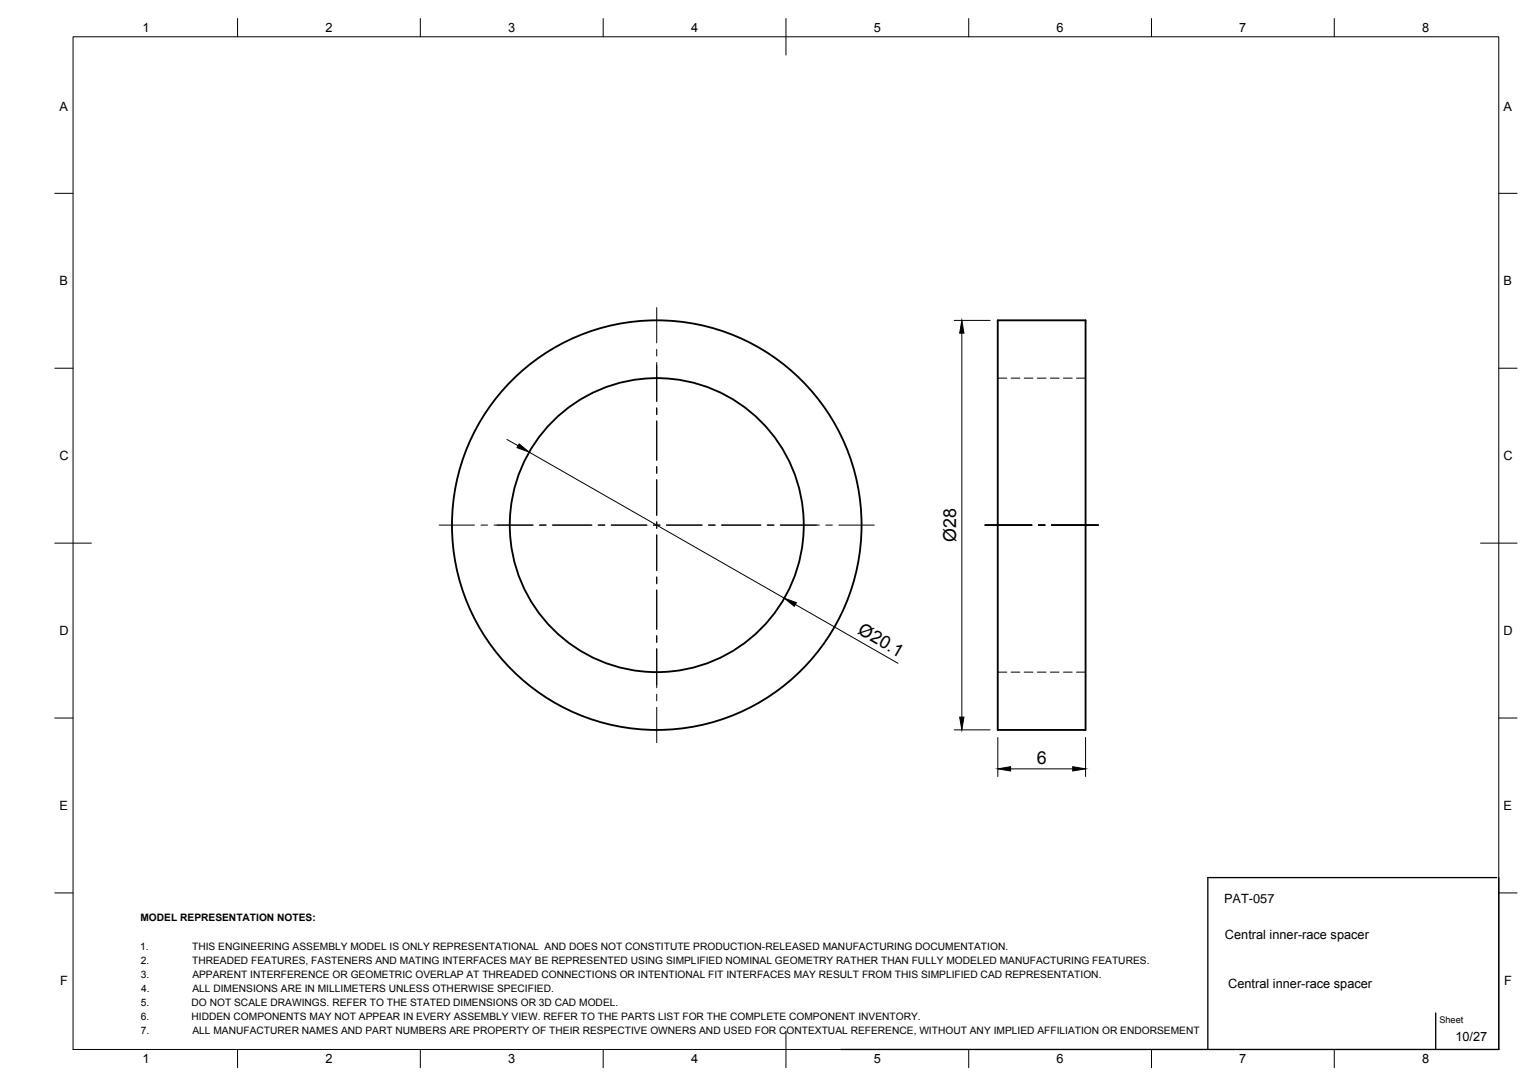
ISO-10303-21;
HEADER;
/* Generated by software containing ST-Developer
 * from STEP Tools, Inc. (www.steptools.com) 
 */

FILE_DESCRIPTION(
/* description */ ('Bearing-mounted hook block'),
/* implementation_level */ '2;1');

FILE_NAME(
/* name */ 'Central inner-race spacer.step',
/* time_stamp */ '2026-10-28T22:30:11-07:00',
/* author */ (''),
/* organization */ (''),
/* preprocessor_version */ 'ST-DEVELOPER v20.2',
/* originating_system */ 'Autodesk Translation Framework v15.17.0.0',
/* authorisation */ '');

FILE_SCHEMA (('AUTOMOTIVE_DESIGN { 1 0 10303 214 3 1 1 }'));
ENDSEC;

DATA;
#10=MECHANICAL_DESIGN_GEOMETRIC_PRESENTATION_REPRESENTATION('',(#328),#7609);
#280=SHAPE_REPRESENTATION_RELATIONSHIP('SRR','None',#7727,#304);
#304=ADVANCED_BREP_SHAPE_REPRESENTATION('',(#360),#7587);
#328=STYLED_ITEM('',(#7917),#360);
#360=MANIFOLD_SOLID_BREP('Body1',#3924);
#447=LINE('',#6319,#677);
#448=LINE('',#6325,#678);
#677=VECTOR('',#5046,1.005);
#678=VECTOR('',#5053,1.4);
#867=CYLINDRICAL_SURFACE('',#4330,1.005);
#868=CYLINDRICAL_SURFACE('',#4333,1.4);
#947=FACE_BOUND('',#1315,.T.);
#948=FACE_BOUND('',#1317,.T.);
#1050=FACE_OUTER_BOUND('',#1312,.T.);
#1051=FACE_OUTER_BOUND('',#1313,.T.);
#1052=FACE_OUTER_BOUND('',#1314,.T.);
#1053=FACE_OUTER_BOUND('',#1316,.T.);
#1312=EDGE_LOOP('',(#2824,#2825,#2826,#2827));
#1313=EDGE_LOOP('',(#2828,#2829,#2830,#2831));
#1314=EDGE_LOOP('',(#2832));
#1315=EDGE_LOOP('',(#2833));
#1316=EDGE_LOOP('',(#2834));
#1317=EDGE_LOOP('',(#2835));
#1607=CIRCLE('',#4331,1.005);
#1608=CIRCLE('',#4332,1.005);
#1609=CIRCLE('',#4334,1.4);
#1610=CIRCLE('',#4335,1.4);
#1856=VERTEX_POINT('',#6316);
#1857=VERTEX_POINT('',#6318);
#1858=VERTEX_POINT('',#6322);
#1859=VERTEX_POINT('',#6324);
#2222=EDGE_CURVE('',#1856,#1856,#1607,.T.);
#2223=EDGE_CURVE('',#1856,#1857,#447,.T.);
#2224=EDGE_CURVE('',#1857,#1857,#1608,.T.);
#2225=EDGE_CURVE('',#1858,#1858,#1609,.T.);
#2226=EDGE_CURVE('',#1858,#1859,#448,.T.);
#2227=EDGE_CURVE('',#1859,#1859,#1610,.T.);
#2824=ORIENTED_EDGE('',*,*,#2222,.F.);
#2825=ORIENTED_EDGE('',*,*,#2223,.T.);
#2826=ORIENTED_EDGE('',*,*,#2224,.T.);
#2827=ORIENTED_EDGE('',*,*,#2223,.F.);
#2828=ORIENTED_EDGE('',*,*,#2225,.F.);
#2829=ORIENTED_EDGE('',*,*,#2226,.T.);
#2830=ORIENTED_EDGE('',*,*,#2227,.T.);
#2831=ORIENTED_EDGE('',*,*,#2226,.F.);
#2832=ORIENTED_EDGE('',*,*,#2225,.T.);
#2833=ORIENTED_EDGE('',*,*,#2222,.T.);
#2834=ORIENTED_EDGE('',*,*,#2227,.F.);
#2835=ORIENTED_EDGE('',*,*,#2224,.F.);
#3586=PLANE('',#4336);
#3587=PLANE('',#4337);
#3732=ADVANCED_FACE('',(#1050),#867,.F.);
#3733=ADVANCED_FACE('',(#1051),#868,.T.);
#3734=ADVANCED_FACE('',(#1052,#947),#3586,.T.);
#3735=ADVANCED_FACE('',(#1053,#948),#3587,.F.);
#3924=CLOSED_SHELL('',(#3732,#3733,#3734,#3735));
#4329=AXIS2_PLACEMENT_3D('',#6314,#5040,#5041);
#4330=AXIS2_PLACEMENT_3D('',#6315,#5042,#5043);
#4331=AXIS2_PLACEMENT_3D('',#6317,#5044,#5045);
#4332=AXIS2_PLACEMENT_3D('',#6320,#5047,#5048);
#4333=AXIS2_PLACEMENT_3D('',#6321,#5049,#5050);
#4334=AXIS2_PLACEMENT_3D('',#6323,#5051,#5052);
#4335=AXIS2_PLACEMENT_3D('',#6326,#5054,#5055);
#4336=AXIS2_PLACEMENT_3D('',#6327,#5056,#5057);
#4337=AXIS2_PLACEMENT_3D('',#6328,#5058,#5059);
#5040=DIRECTION('axis',(0.,0.,1.));
#5041=DIRECTION('refdir',(1.,0.,0.));
#5042=DIRECTION('center_axis',(0.,1.,0.));
#5043=DIRECTION('ref_axis',(1.,0.,0.));
#5044=DIRECTION('center_axis',(0.,-1.,0.));
#5045=DIRECTION('ref_axis',(1.,0.,0.));
#5046=DIRECTION('',(0.,-1.,0.));
#5047=DIRECTION('center_axis',(0.,-1.,0.));
#5048=DIRECTION('ref_axis',(1.,0.,0.));
#5049=DIRECTION('center_axis',(0.,1.,0.));
#5050=DIRECTION('ref_axis',(1.,0.,0.));
#5051=DIRECTION('center_axis',(0.,1.,0.));
#5052=DIRECTION('ref_axis',(1.,0.,0.));
#5053=DIRECTION('',(0.,-1.,0.));
#5054=DIRECTION('center_axis',(0.,1.,0.));
#5055=DIRECTION('ref_axis',(1.,0.,0.));
#5056=DIRECTION('center_axis',(0.,1.,0.));
#5057=DIRECTION('ref_axis',(1.,0.,0.));
#5058=DIRECTION('center_axis',(0.,1.,0.));
#5059=DIRECTION('ref_axis',(1.,0.,0.));
#6314=CARTESIAN_POINT('',(0.,0.,0.));
#6315=CARTESIAN_POINT('Origin',(0.,-0.3,12.));
#6316=CARTESIAN_POINT('',(-1.005,0.3,12.));
#6317=CARTESIAN_POINT('Origin',(0.,0.3,12.));
#6318=CARTESIAN_POINT('',(-1.005,-0.3,12.));
#6319=CARTESIAN_POINT('',(-1.005,-0.3,12.));
#6320=CARTESIAN_POINT('Origin',(0.,-0.3,12.));
#6321=CARTESIAN_POINT('Origin',(0.,-0.3,12.));
#6322=CARTESIAN_POINT('',(-1.4,0.3,12.));
#6323=CARTESIAN_POINT('Origin',(0.,0.3,12.));
#6324=CARTESIAN_POINT('',(-1.4,-0.3,12.));
#6325=CARTESIAN_POINT('',(-1.4,-0.3,12.));
#6326=CARTESIAN_POINT('Origin',(0.,-0.3,12.));
#6327=CARTESIAN_POINT('Origin',(0.,0.3,12.));
#6328=CARTESIAN_POINT('Origin',(0.,-0.3,12.));
#7557=UNCERTAINTY_MEASURE_WITH_UNIT(LENGTH_MEASURE(0.001),#7610,
'DISTANCE_ACCURACY_VALUE',
'Maximum model space distance between geometric entities at asserted c
onnectivities');
#7579=UNCERTAINTY_MEASURE_WITH_UNIT(LENGTH_MEASURE(0.001),#7610,
'DISTANCE_ACCURACY_VALUE',
'Maximum model space distance between geometric entities at asserted c
onnectivities');
#7587=(
GEOMETRIC_REPRESENTATION_CONTEXT(3)
GLOBAL_UNCERTAINTY_ASSIGNED_CONTEXT((#7557))
GLOBAL_UNIT_ASSIGNED_CONTEXT((#7610,#7612,#7613))
REPRESENTATION_CONTEXT('','3D')
);
#7609=(
GEOMETRIC_REPRESENTATION_CONTEXT(3)
GLOBAL_UNCERTAINTY_ASSIGNED_CONTEXT((#7579))
GLOBAL_UNIT_ASSIGNED_CONTEXT((#7610,#7612,#7613))
REPRESENTATION_CONTEXT('','3D')
);
#7610=(
LENGTH_UNIT()
NAMED_UNIT(*)
SI_UNIT(.CENTI.,.METRE.)
);
#7612=(
NAMED_UNIT(*)
PLANE_ANGLE_UNIT()
SI_UNIT($,.RADIAN.)
);
#7613=(
NAMED_UNIT(*)
SI_UNIT($,.STERADIAN.)
SOLID_ANGLE_UNIT()
);
#7621=SHAPE_DEFINITION_REPRESENTATION(#7650,#7727);
#7650=PRODUCT_DEFINITION_SHAPE('',$,#7757);
#7727=SHAPE_REPRESENTATION('',(#4329),#7587);
#7749=PRODUCT_DEFINITION_CONTEXT('part definition',#7838,'design');
#7757=PRODUCT_DEFINITION('Central inner-race spacer',
'Central inner-race spacer',#7786,#7749);
#7786=PRODUCT_DEFINITION_FORMATION('',$,#7847);
#7838=APPLICATION_CONTEXT(
'Core Data for Automotive Mechanical Design Process');
#7839=PRODUCT_CONTEXT('part definition',#7838,'mechanical');
#7847=PRODUCT('Central inner-race spacer','Central inner-race spacer',
'Central inner-race spacer',(#7839));
#7911=COLOUR_RGB('Light Blue',0.38,0.62,0.78);
#7912=FILL_AREA_STYLE_COLOUR('',#7911);
#7913=FILL_AREA_STYLE('',(#7912));
#7914=SURFACE_STYLE_FILL_AREA(#7913);
#7915=SURFACE_SIDE_STYLE('',(#7914));
#7916=SURFACE_STYLE_USAGE(.BOTH.,#7915);
#7917=PRESENTATION_STYLE_ASSIGNMENT((#7916));
ENDSEC;
END-ISO-10303-21;
